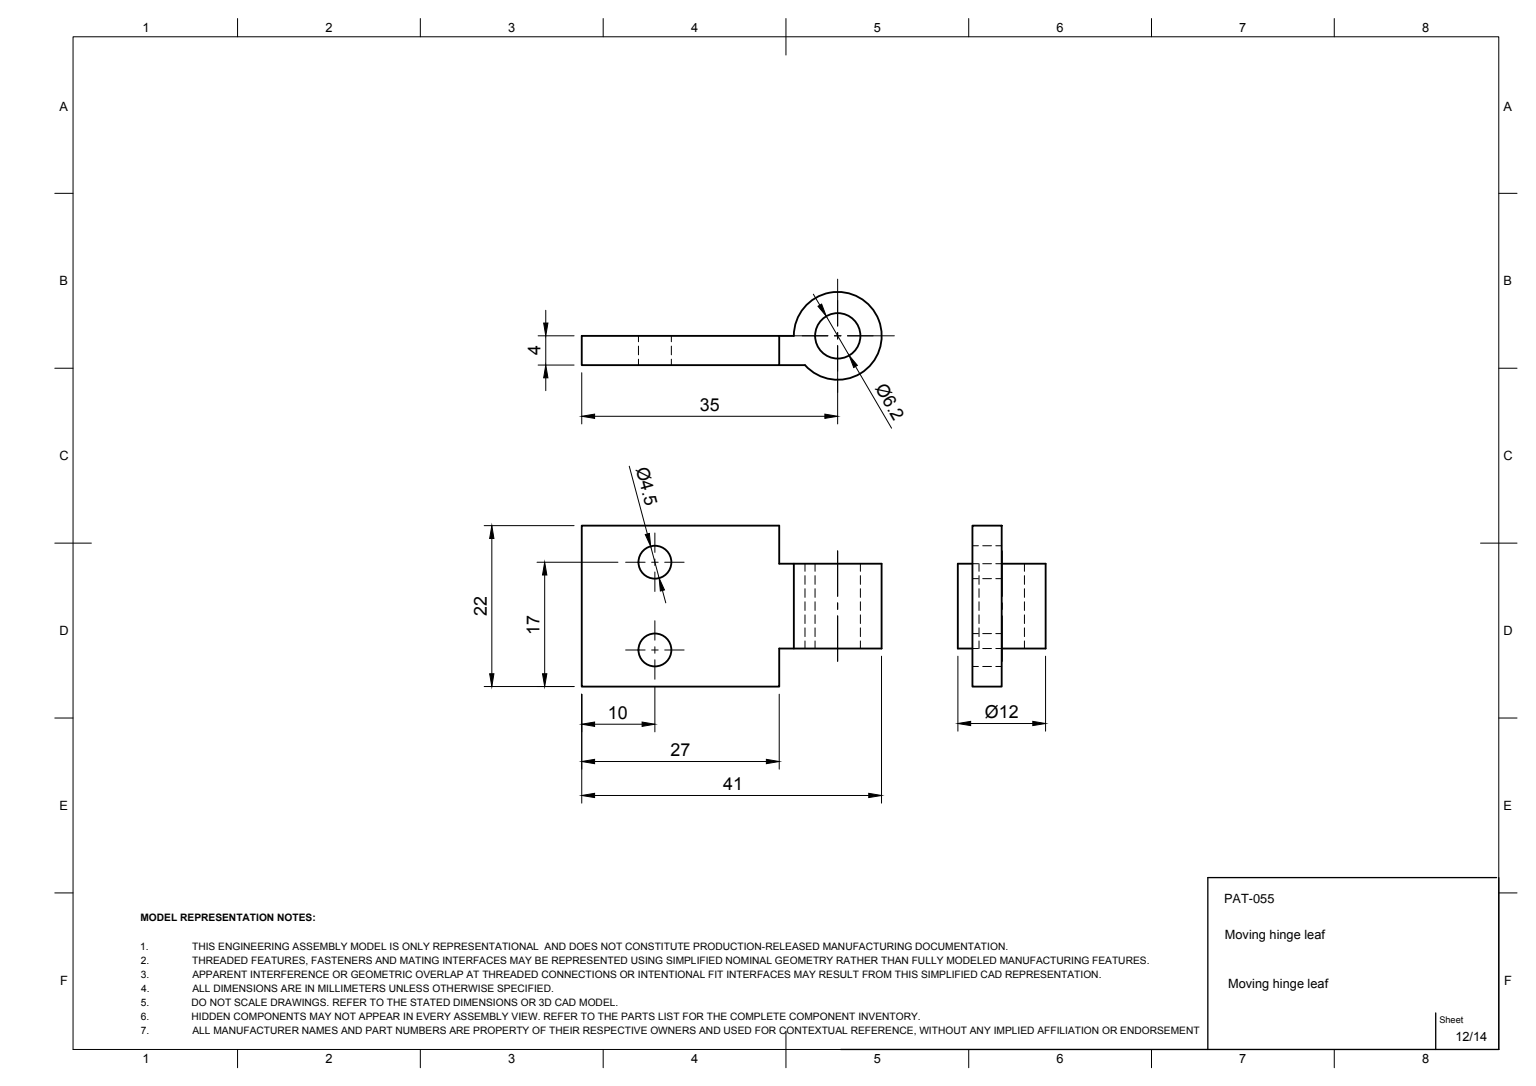
ISO-10303-21;
HEADER;
/* Generated by software containing ST-Developer
 * from STEP Tools, Inc. (www.steptools.com) 
 */

FILE_DESCRIPTION(
/* description */ ('Hinged panel with latch'),
/* implementation_level */ '2;1');

FILE_NAME(
/* name */ 'Moving hinge leaf.step',
/* time_stamp */ '2026-10-27T20:36:01-07:00',
/* author */ (''),
/* organization */ (''),
/* preprocessor_version */ 'ST-DEVELOPER v20.2',
/* originating_system */ 'Autodesk Translation Framework v15.17.0.0',
/* authorisation */ '');

FILE_SCHEMA (('AUTOMOTIVE_DESIGN { 1 0 10303 214 3 1 1 }'));
ENDSEC;

DATA;
#10=MECHANICAL_DESIGN_GEOMETRIC_PRESENTATION_REPRESENTATION('',(#305),#6743);
#273=SHAPE_REPRESENTATION_RELATIONSHIP('SRR','None',#6849,#289);
#289=ADVANCED_BREP_SHAPE_REPRESENTATION('',(#320),#6735);
#305=STYLED_ITEM('',(#6989),#320);
#320=MANIFOLD_SOLID_BREP('Body1',#3808);
#356=FACE_BOUND('',#894,.T.);
#357=FACE_BOUND('',#896,.T.);
#358=FACE_BOUND('',#897,.T.);
#359=FACE_BOUND('',#899,.T.);
#360=FACE_BOUND('',#900,.T.);
#361=FACE_BOUND('',#903,.T.);
#468=PLANE('',#4197);
#469=PLANE('',#4198);
#470=PLANE('',#4199);
#471=PLANE('',#4200);
#472=PLANE('',#4201);
#473=PLANE('',#4202);
#474=PLANE('',#4204);
#475=PLANE('',#4205);
#476=PLANE('',#4208);
#648=FACE_OUTER_BOUND('',#885,.T.);
#649=FACE_OUTER_BOUND('',#886,.T.);
#650=FACE_OUTER_BOUND('',#887,.T.);
#651=FACE_OUTER_BOUND('',#888,.T.);
#652=FACE_OUTER_BOUND('',#889,.T.);
#653=FACE_OUTER_BOUND('',#890,.T.);
#654=FACE_OUTER_BOUND('',#891,.T.);
#655=FACE_OUTER_BOUND('',#892,.T.);
#656=FACE_OUTER_BOUND('',#893,.T.);
#657=FACE_OUTER_BOUND('',#895,.T.);
#658=FACE_OUTER_BOUND('',#898,.T.);
#659=FACE_OUTER_BOUND('',#901,.T.);
#660=FACE_OUTER_BOUND('',#902,.T.);
#885=EDGE_LOOP('',(#3216,#3217,#3218,#3219));
#886=EDGE_LOOP('',(#3220,#3221,#3222,#3223));
#887=EDGE_LOOP('',(#3224,#3225,#3226,#3227));
#888=EDGE_LOOP('',(#3228,#3229,#3230,#3231));
#889=EDGE_LOOP('',(#3232,#3233,#3234,#3235));
#890=EDGE_LOOP('',(#3236,#3237,#3238,#3239));
#891=EDGE_LOOP('',(#3240,#3241,#3242,#3243));
#892=EDGE_LOOP('',(#3244,#3245,#3246,#3247));
#893=EDGE_LOOP('',(#3248,#3249,#3250,#3251));
#894=EDGE_LOOP('',(#3252));
#895=EDGE_LOOP('',(#3253,#3254,#3255,#3256,#3257,#3258,#3259,#3260));
#896=EDGE_LOOP('',(#3261));
#897=EDGE_LOOP('',(#3262));
#898=EDGE_LOOP('',(#3263,#3264,#3265,#3266,#3267,#3268,#3269,#3270));
#899=EDGE_LOOP('',(#3271));
#900=EDGE_LOOP('',(#3272));
#901=EDGE_LOOP('',(#3273,#3274,#3275,#3276));
#902=EDGE_LOOP('',(#3277,#3278,#3279,#3280));
#903=EDGE_LOOP('',(#3281));
#1233=LINE('',#6242,#1591);
#1234=LINE('',#6248,#1592);
#1235=LINE('',#6254,#1593);
#1236=LINE('',#6259,#1594);
#1237=LINE('',#6261,#1595);
#1238=LINE('',#6263,#1596);
#1239=LINE('',#6264,#1597);
#1240=LINE('',#6268,#1598);
#1241=LINE('',#6270,#1599);
#1242=LINE('',#6272,#1600);
#1243=LINE('',#6273,#1601);
#1244=LINE('',#6276,#1602);
#1245=LINE('',#6278,#1603);
#1246=LINE('',#6279,#1604);
#1247=LINE('',#6282,#1605);
#1248=LINE('',#6284,#1606);
#1249=LINE('',#6285,#1607);
#1250=LINE('',#6287,#1608);
#1251=LINE('',#6288,#1609);
#1252=LINE('',#6291,#1610);
#1253=LINE('',#6294,#1611);
#1254=LINE('',#6297,#1612);
#1255=LINE('',#6298,#1613);
#1256=LINE('',#6301,#1614);
#1257=LINE('',#6302,#1615);
#1591=VECTOR('',#5007,0.225);
#1592=VECTOR('',#5014,0.225);
#1593=VECTOR('',#5021,0.31);
#1594=VECTOR('',#5026,1.);
#1595=VECTOR('',#5027,1.);
#1596=VECTOR('',#5028,1.);
#1597=VECTOR('',#5029,1.);
#1598=VECTOR('',#5032,1.);
#1599=VECTOR('',#5033,1.);
#1600=VECTOR('',#5034,1.);
#1601=VECTOR('',#5035,1.);
#1602=VECTOR('',#5038,1.);
#1603=VECTOR('',#5039,1.);
#1604=VECTOR('',#5040,1.);
#1605=VECTOR('',#5043,1.);
#1606=VECTOR('',#5044,1.);
#1607=VECTOR('',#5045,1.);
#1608=VECTOR('',#5048,1.);
#1609=VECTOR('',#5049,1.);
#1610=VECTOR('',#5052,1.);
#1611=VECTOR('',#5055,1.);
#1612=VECTOR('',#5058,1.);
#1613=VECTOR('',#5059,1.);
#1614=VECTOR('',#5062,1.);
#1615=VECTOR('',#5063,1.);
#1752=CIRCLE('',#4189,0.225);
#1753=CIRCLE('',#4190,0.225);
#1754=CIRCLE('',#4192,0.225);
#1755=CIRCLE('',#4193,0.225);
#1756=CIRCLE('',#4195,0.31);
#1757=CIRCLE('',#4196,0.31);
#1758=CIRCLE('',#4203,0.6);
#1759=CIRCLE('',#4207,0.6);
#1998=VERTEX_POINT('',#6239);
#1999=VERTEX_POINT('',#6241);
#2000=VERTEX_POINT('',#6245);
#2001=VERTEX_POINT('',#6247);
#2002=VERTEX_POINT('',#6251);
#2003=VERTEX_POINT('',#6253);
#2004=VERTEX_POINT('',#6257);
#2005=VERTEX_POINT('',#6258);
#2006=VERTEX_POINT('',#6260);
#2007=VERTEX_POINT('',#6262);
#2008=VERTEX_POINT('',#6266);
#2009=VERTEX_POINT('',#6267);
#2010=VERTEX_POINT('',#6269);
#2011=VERTEX_POINT('',#6271);
#2012=VERTEX_POINT('',#6275);
#2013=VERTEX_POINT('',#6277);
#2014=VERTEX_POINT('',#6281);
#2015=VERTEX_POINT('',#6283);
#2016=VERTEX_POINT('',#6290);
#2017=VERTEX_POINT('',#6292);
#2018=VERTEX_POINT('',#6296);
#2019=VERTEX_POINT('',#6300);
#2420=EDGE_CURVE('',#1998,#1998,#1752,.T.);
#2421=EDGE_CURVE('',#1998,#1999,#1233,.T.);
#2422=EDGE_CURVE('',#1999,#1999,#1753,.T.);
#2423=EDGE_CURVE('',#2000,#2000,#1754,.T.);
#2424=EDGE_CURVE('',#2000,#2001,#1234,.T.);
#2425=EDGE_CURVE('',#2001,#2001,#1755,.T.);
#2426=EDGE_CURVE('',#2002,#2002,#1756,.T.);
#2427=EDGE_CURVE('',#2002,#2003,#1235,.T.);
#2428=EDGE_CURVE('',#2003,#2003,#1757,.T.);
#2429=EDGE_CURVE('',#2004,#2005,#1236,.T.);
#2430=EDGE_CURVE('',#2006,#2004,#1237,.T.);
#2431=EDGE_CURVE('',#2006,#2007,#1238,.T.);
#2432=EDGE_CURVE('',#2005,#2007,#1239,.T.);
#2433=EDGE_CURVE('',#2008,#2009,#1240,.T.);
#2434=EDGE_CURVE('',#2010,#2008,#1241,.T.);
#2435=EDGE_CURVE('',#2011,#2010,#1242,.T.);
#2436=EDGE_CURVE('',#2009,#2011,#1243,.T.);
#2437=EDGE_CURVE('',#2011,#2012,#1244,.T.);
#2438=EDGE_CURVE('',#2013,#2010,#1245,.T.);
#2439=EDGE_CURVE('',#2012,#2013,#1246,.T.);
#2440=EDGE_CURVE('',#2012,#2014,#1247,.T.);
#2441=EDGE_CURVE('',#2015,#2013,#1248,.T.);
#2442=EDGE_CURVE('',#2014,#2015,#1249,.T.);
#2443=EDGE_CURVE('',#2014,#2006,#1250,.T.);
#2444=EDGE_CURVE('',#2007,#2015,#1251,.T.);
#2445=EDGE_CURVE('',#2016,#2009,#1252,.T.);
#2446=EDGE_CURVE('',#2017,#2016,#1758,.T.);
#2447=EDGE_CURVE('',#2008,#2017,#1253,.T.);
#2448=EDGE_CURVE('',#2004,#2018,#1254,.T.);
#2449=EDGE_CURVE('',#2016,#2018,#1255,.T.);
#2450=EDGE_CURVE('',#2019,#2017,#1256,.T.);
#2451=EDGE_CURVE('',#2019,#2005,#1257,.T.);
#2452=EDGE_CURVE('',#2019,#2018,#1759,.T.);
#3216=ORIENTED_EDGE('',*,*,#2420,.F.);
#3217=ORIENTED_EDGE('',*,*,#2421,.T.);
#3218=ORIENTED_EDGE('',*,*,#2422,.F.);
#3219=ORIENTED_EDGE('',*,*,#2421,.F.);
#3220=ORIENTED_EDGE('',*,*,#2423,.F.);
#3221=ORIENTED_EDGE('',*,*,#2424,.T.);
#3222=ORIENTED_EDGE('',*,*,#2425,.F.);
#3223=ORIENTED_EDGE('',*,*,#2424,.F.);
#3224=ORIENTED_EDGE('',*,*,#2426,.F.);
#3225=ORIENTED_EDGE('',*,*,#2427,.T.);
#3226=ORIENTED_EDGE('',*,*,#2428,.F.);
#3227=ORIENTED_EDGE('',*,*,#2427,.F.);
#3228=ORIENTED_EDGE('',*,*,#2429,.F.);
#3229=ORIENTED_EDGE('',*,*,#2430,.F.);
#3230=ORIENTED_EDGE('',*,*,#2431,.T.);
#3231=ORIENTED_EDGE('',*,*,#2432,.F.);
#3232=ORIENTED_EDGE('',*,*,#2433,.F.);
#3233=ORIENTED_EDGE('',*,*,#2434,.F.);
#3234=ORIENTED_EDGE('',*,*,#2435,.F.);
#3235=ORIENTED_EDGE('',*,*,#2436,.F.);
#3236=ORIENTED_EDGE('',*,*,#2437,.F.);
#3237=ORIENTED_EDGE('',*,*,#2435,.T.);
#3238=ORIENTED_EDGE('',*,*,#2438,.F.);
#3239=ORIENTED_EDGE('',*,*,#2439,.F.);
#3240=ORIENTED_EDGE('',*,*,#2440,.F.);
#3241=ORIENTED_EDGE('',*,*,#2439,.T.);
#3242=ORIENTED_EDGE('',*,*,#2441,.F.);
#3243=ORIENTED_EDGE('',*,*,#2442,.F.);
#3244=ORIENTED_EDGE('',*,*,#2443,.F.);
#3245=ORIENTED_EDGE('',*,*,#2442,.T.);
#3246=ORIENTED_EDGE('',*,*,#2444,.F.);
#3247=ORIENTED_EDGE('',*,*,#2431,.F.);
#3248=ORIENTED_EDGE('',*,*,#2433,.T.);
#3249=ORIENTED_EDGE('',*,*,#2445,.F.);
#3250=ORIENTED_EDGE('',*,*,#2446,.F.);
#3251=ORIENTED_EDGE('',*,*,#2447,.F.);
#3252=ORIENTED_EDGE('',*,*,#2426,.T.);
#3253=ORIENTED_EDGE('',*,*,#2448,.T.);
#3254=ORIENTED_EDGE('',*,*,#2449,.F.);
#3255=ORIENTED_EDGE('',*,*,#2445,.T.);
#3256=ORIENTED_EDGE('',*,*,#2436,.T.);
#3257=ORIENTED_EDGE('',*,*,#2437,.T.);
#3258=ORIENTED_EDGE('',*,*,#2440,.T.);
#3259=ORIENTED_EDGE('',*,*,#2443,.T.);
#3260=ORIENTED_EDGE('',*,*,#2430,.T.);
#3261=ORIENTED_EDGE('',*,*,#2420,.T.);
#3262=ORIENTED_EDGE('',*,*,#2423,.T.);
#3263=ORIENTED_EDGE('',*,*,#2447,.T.);
#3264=ORIENTED_EDGE('',*,*,#2450,.F.);
#3265=ORIENTED_EDGE('',*,*,#2451,.T.);
#3266=ORIENTED_EDGE('',*,*,#2432,.T.);
#3267=ORIENTED_EDGE('',*,*,#2444,.T.);
#3268=ORIENTED_EDGE('',*,*,#2441,.T.);
#3269=ORIENTED_EDGE('',*,*,#2438,.T.);
#3270=ORIENTED_EDGE('',*,*,#2434,.T.);
#3271=ORIENTED_EDGE('',*,*,#2422,.T.);
#3272=ORIENTED_EDGE('',*,*,#2425,.T.);
#3273=ORIENTED_EDGE('',*,*,#2449,.T.);
#3274=ORIENTED_EDGE('',*,*,#2452,.F.);
#3275=ORIENTED_EDGE('',*,*,#2450,.T.);
#3276=ORIENTED_EDGE('',*,*,#2446,.T.);
#3277=ORIENTED_EDGE('',*,*,#2429,.T.);
#3278=ORIENTED_EDGE('',*,*,#2451,.F.);
#3279=ORIENTED_EDGE('',*,*,#2452,.T.);
#3280=ORIENTED_EDGE('',*,*,#2448,.F.);
#3281=ORIENTED_EDGE('',*,*,#2428,.T.);
#3579=CYLINDRICAL_SURFACE('',#4188,0.225);
#3580=CYLINDRICAL_SURFACE('',#4191,0.225);
#3581=CYLINDRICAL_SURFACE('',#4194,0.31);
#3582=CYLINDRICAL_SURFACE('',#4206,0.6);
#3717=ADVANCED_FACE('',(#648),#3579,.F.);
#3718=ADVANCED_FACE('',(#649),#3580,.F.);
#3719=ADVANCED_FACE('',(#650),#3581,.F.);
#3720=ADVANCED_FACE('',(#651),#468,.T.);
#3721=ADVANCED_FACE('',(#652),#469,.T.);
#3722=ADVANCED_FACE('',(#653),#470,.T.);
#3723=ADVANCED_FACE('',(#654),#471,.T.);
#3724=ADVANCED_FACE('',(#655),#472,.T.);
#3725=ADVANCED_FACE('',(#656,#356),#473,.F.);
#3726=ADVANCED_FACE('',(#657,#357,#358),#474,.F.);
#3727=ADVANCED_FACE('',(#658,#359,#360),#475,.T.);
#3728=ADVANCED_FACE('',(#659),#3582,.T.);
#3729=ADVANCED_FACE('',(#660,#361),#476,.T.);
#3808=CLOSED_SHELL('',(#3717,#3718,#3719,#3720,#3721,#3722,#3723,#3724,
#3725,#3726,#3727,#3728,#3729));
#4187=AXIS2_PLACEMENT_3D('',#6237,#5001,#5002);
#4188=AXIS2_PLACEMENT_3D('',#6238,#5003,#5004);
#4189=AXIS2_PLACEMENT_3D('',#6240,#5005,#5006);
#4190=AXIS2_PLACEMENT_3D('',#6243,#5008,#5009);
#4191=AXIS2_PLACEMENT_3D('',#6244,#5010,#5011);
#4192=AXIS2_PLACEMENT_3D('',#6246,#5012,#5013);
#4193=AXIS2_PLACEMENT_3D('',#6249,#5015,#5016);
#4194=AXIS2_PLACEMENT_3D('',#6250,#5017,#5018);
#4195=AXIS2_PLACEMENT_3D('',#6252,#5019,#5020);
#4196=AXIS2_PLACEMENT_3D('',#6255,#5022,#5023);
#4197=AXIS2_PLACEMENT_3D('',#6256,#5024,#5025);
#4198=AXIS2_PLACEMENT_3D('',#6265,#5030,#5031);
#4199=AXIS2_PLACEMENT_3D('',#6274,#5036,#5037);
#4200=AXIS2_PLACEMENT_3D('',#6280,#5041,#5042);
#4201=AXIS2_PLACEMENT_3D('',#6286,#5046,#5047);
#4202=AXIS2_PLACEMENT_3D('',#6289,#5050,#5051);
#4203=AXIS2_PLACEMENT_3D('',#6293,#5053,#5054);
#4204=AXIS2_PLACEMENT_3D('',#6295,#5056,#5057);
#4205=AXIS2_PLACEMENT_3D('',#6299,#5060,#5061);
#4206=AXIS2_PLACEMENT_3D('',#6303,#5064,#5065);
#4207=AXIS2_PLACEMENT_3D('',#6304,#5066,#5067);
#4208=AXIS2_PLACEMENT_3D('',#6305,#5068,#5069);
#5001=DIRECTION('axis',(0.,0.,1.));
#5002=DIRECTION('refdir',(1.,0.,0.));
#5003=DIRECTION('center_axis',(0.,1.,0.));
#5004=DIRECTION('ref_axis',(1.,0.,0.));
#5005=DIRECTION('center_axis',(0.,1.,0.));
#5006=DIRECTION('ref_axis',(1.,0.,0.));
#5007=DIRECTION('',(0.,1.,0.));
#5008=DIRECTION('center_axis',(0.,-1.,0.));
#5009=DIRECTION('ref_axis',(1.,0.,0.));
#5010=DIRECTION('center_axis',(0.,1.,0.));
#5011=DIRECTION('ref_axis',(1.,0.,0.));
#5012=DIRECTION('center_axis',(0.,1.,0.));
#5013=DIRECTION('ref_axis',(1.,0.,0.));
#5014=DIRECTION('',(0.,1.,0.));
#5015=DIRECTION('center_axis',(0.,-1.,0.));
#5016=DIRECTION('ref_axis',(1.,0.,0.));
#5017=DIRECTION('center_axis',(0.,0.,1.));
#5018=DIRECTION('ref_axis',(1.,0.,0.));
#5019=DIRECTION('center_axis',(0.,0.,1.));
#5020=DIRECTION('ref_axis',(1.,0.,0.));
#5021=DIRECTION('',(0.,0.,1.));
#5022=DIRECTION('center_axis',(0.,0.,-1.));
#5023=DIRECTION('ref_axis',(1.,0.,0.));
#5024=DIRECTION('center_axis',(-1.,0.,0.));
#5025=DIRECTION('ref_axis',(0.,0.,1.));
#5026=DIRECTION('',(0.,1.,0.));
#5027=DIRECTION('',(0.,0.,-1.));
#5028=DIRECTION('',(0.,1.,0.));
#5029=DIRECTION('',(0.,0.,1.));
#5030=DIRECTION('center_axis',(-1.,0.,0.));
#5031=DIRECTION('ref_axis',(0.,0.,1.));
#5032=DIRECTION('',(0.,-1.,0.));
#5033=DIRECTION('',(0.,0.,1.));
#5034=DIRECTION('',(0.,1.,0.));
#5035=DIRECTION('',(0.,0.,-1.));
#5036=DIRECTION('center_axis',(0.,0.,-1.));
#5037=DIRECTION('ref_axis',(-1.,0.,0.));
#5038=DIRECTION('',(1.,0.,0.));
#5039=DIRECTION('',(-1.,0.,0.));
#5040=DIRECTION('',(0.,1.,0.));
#5041=DIRECTION('center_axis',(1.,0.,0.));
#5042=DIRECTION('ref_axis',(0.,0.,-1.));
#5043=DIRECTION('',(0.,0.,1.));
#5044=DIRECTION('',(0.,0.,-1.));
#5045=DIRECTION('',(0.,1.,0.));
#5046=DIRECTION('center_axis',(0.,0.,1.));
#5047=DIRECTION('ref_axis',(1.,0.,0.));
#5048=DIRECTION('',(-1.,0.,0.));
#5049=DIRECTION('',(1.,0.,0.));
#5050=DIRECTION('center_axis',(0.,0.,1.));
#5051=DIRECTION('ref_axis',(1.,0.,0.));
#5052=DIRECTION('',(1.,0.,0.));
#5053=DIRECTION('center_axis',(0.,0.,1.));
#5054=DIRECTION('ref_axis',(1.,0.,0.));
#5055=DIRECTION('',(-1.,0.,0.));
#5056=DIRECTION('center_axis',(0.,1.,0.));
#5057=DIRECTION('ref_axis',(1.,0.,0.));
#5058=DIRECTION('',(-1.,0.,0.));
#5059=DIRECTION('',(0.,0.,1.));
#5060=DIRECTION('center_axis',(0.,1.,0.));
#5061=DIRECTION('ref_axis',(0.,0.,1.));
#5062=DIRECTION('',(0.,0.,-1.));
#5063=DIRECTION('',(1.,0.,0.));
#5064=DIRECTION('center_axis',(0.,0.,1.));
#5065=DIRECTION('ref_axis',(-0.934172358962716,0.35682208977309,0.));
#5066=DIRECTION('center_axis',(0.,0.,1.));
#5067=DIRECTION('ref_axis',(1.,0.,0.));
#5068=DIRECTION('center_axis',(0.,0.,1.));
#5069=DIRECTION('ref_axis',(1.,0.,0.));
#6237=CARTESIAN_POINT('',(0.,0.,0.));
#6238=CARTESIAN_POINT('Origin',(4.5,-2.3,6.));
#6239=CARTESIAN_POINT('',(4.275,-2.2,6.));
#6240=CARTESIAN_POINT('Origin',(4.5,-2.2,6.));
#6241=CARTESIAN_POINT('',(4.275,-1.8,6.));
#6242=CARTESIAN_POINT('',(4.275,-2.3,6.));
#6243=CARTESIAN_POINT('Origin',(4.5,-1.8,6.));
#6244=CARTESIAN_POINT('Origin',(4.5,-2.3,7.2));
#6245=CARTESIAN_POINT('',(4.275,-2.2,7.2));
#6246=CARTESIAN_POINT('Origin',(4.5,-2.2,7.2));
#6247=CARTESIAN_POINT('',(4.275,-1.8,7.2));
#6248=CARTESIAN_POINT('',(4.275,-2.3,7.2));
#6249=CARTESIAN_POINT('Origin',(4.5,-1.8,7.2));
#6250=CARTESIAN_POINT('Origin',(2.,-1.8,6.));
#6251=CARTESIAN_POINT('',(1.69,-1.8,6.02));
#6252=CARTESIAN_POINT('Origin',(2.,-1.8,6.02));
#6253=CARTESIAN_POINT('',(1.69,-1.8,7.18));
#6254=CARTESIAN_POINT('',(1.69,-1.8,6.));
#6255=CARTESIAN_POINT('Origin',(2.,-1.8,7.18));
#6256=CARTESIAN_POINT('Origin',(2.8,-2.2,5.5));
#6257=CARTESIAN_POINT('',(2.8,-2.2,7.18));
#6258=CARTESIAN_POINT('',(2.8,-1.8,7.18));
#6259=CARTESIAN_POINT('',(2.8,-2.,7.18));
#6260=CARTESIAN_POINT('',(2.8,-2.2,7.7));
#6261=CARTESIAN_POINT('',(2.8,-2.2,7.7));
#6262=CARTESIAN_POINT('',(2.8,-1.8,7.7));
#6263=CARTESIAN_POINT('',(2.8,-2.2,7.7));
#6264=CARTESIAN_POINT('',(2.8,-1.8,7.7));
#6265=CARTESIAN_POINT('Origin',(2.8,-2.2,5.5));
#6266=CARTESIAN_POINT('',(2.8,-1.8,6.02));
#6267=CARTESIAN_POINT('',(2.8,-2.2,6.02));
#6268=CARTESIAN_POINT('',(2.8,-2.,6.02));
#6269=CARTESIAN_POINT('',(2.8,-1.8,5.5));
#6270=CARTESIAN_POINT('',(2.8,-1.8,7.7));
#6271=CARTESIAN_POINT('',(2.8,-2.2,5.5));
#6272=CARTESIAN_POINT('',(2.8,-2.2,5.5));
#6273=CARTESIAN_POINT('',(2.8,-2.2,7.7));
#6274=CARTESIAN_POINT('Origin',(5.5,-2.2,5.5));
#6275=CARTESIAN_POINT('',(5.5,-2.2,5.5));
#6276=CARTESIAN_POINT('',(2.8,-2.2,5.5));
#6277=CARTESIAN_POINT('',(5.5,-1.8,5.5));
#6278=CARTESIAN_POINT('',(2.8,-1.8,5.5));
#6279=CARTESIAN_POINT('',(5.5,-2.2,5.5));
#6280=CARTESIAN_POINT('Origin',(5.5,-2.2,7.7));
#6281=CARTESIAN_POINT('',(5.5,-2.2,7.7));
#6282=CARTESIAN_POINT('',(5.5,-2.2,5.5));
#6283=CARTESIAN_POINT('',(5.5,-1.8,7.7));
#6284=CARTESIAN_POINT('',(5.5,-1.8,5.5));
#6285=CARTESIAN_POINT('',(5.5,-2.2,7.7));
#6286=CARTESIAN_POINT('Origin',(2.8,-2.2,7.7));
#6287=CARTESIAN_POINT('',(5.5,-2.2,7.7));
#6288=CARTESIAN_POINT('',(5.5,-1.8,7.7));
#6289=CARTESIAN_POINT('Origin',(2.,-1.8,6.02));
#6290=CARTESIAN_POINT('',(2.44721359549996,-2.2,6.02));
#6291=CARTESIAN_POINT('',(2.,-2.2,6.02));
#6292=CARTESIAN_POINT('',(2.6,-1.8,6.02));
#6293=CARTESIAN_POINT('Origin',(2.,-1.8,6.02));
#6294=CARTESIAN_POINT('',(2.,-1.8,6.02));
#6295=CARTESIAN_POINT('Origin',(2.5,-2.2,6.6));
#6296=CARTESIAN_POINT('',(2.44721359549996,-2.2,7.18));
#6297=CARTESIAN_POINT('',(3.,-2.2,7.18));
#6298=CARTESIAN_POINT('',(2.44721359549996,-2.2,6.02));
#6299=CARTESIAN_POINT('Origin',(2.5,-1.8,6.6));
#6300=CARTESIAN_POINT('',(2.6,-1.8,7.18));
#6301=CARTESIAN_POINT('',(2.6,-1.8,6.02));
#6302=CARTESIAN_POINT('',(3.,-1.8,7.18));
#6303=CARTESIAN_POINT('Origin',(2.,-1.8,6.02));
#6304=CARTESIAN_POINT('Origin',(2.,-1.8,7.18));
#6305=CARTESIAN_POINT('Origin',(2.,-1.8,7.18));
#6714=UNCERTAINTY_MEASURE_WITH_UNIT(LENGTH_MEASURE(0.001),#6744,
'DISTANCE_ACCURACY_VALUE',
'Maximum model space distance between geometric entities at asserted c
onnectivities');
#6722=UNCERTAINTY_MEASURE_WITH_UNIT(LENGTH_MEASURE(0.001),#6744,
'DISTANCE_ACCURACY_VALUE',
'Maximum model space distance between geometric entities at asserted c
onnectivities');
#6735=(
GEOMETRIC_REPRESENTATION_CONTEXT(3)
GLOBAL_UNCERTAINTY_ASSIGNED_CONTEXT((#6714))
GLOBAL_UNIT_ASSIGNED_CONTEXT((#6744,#6746,#6747))
REPRESENTATION_CONTEXT('','3D')
);
#6743=(
GEOMETRIC_REPRESENTATION_CONTEXT(3)
GLOBAL_UNCERTAINTY_ASSIGNED_CONTEXT((#6722))
GLOBAL_UNIT_ASSIGNED_CONTEXT((#6744,#6746,#6747))
REPRESENTATION_CONTEXT('','3D')
);
#6744=(
LENGTH_UNIT()
NAMED_UNIT(*)
SI_UNIT(.CENTI.,.METRE.)
);
#6746=(
NAMED_UNIT(*)
PLANE_ANGLE_UNIT()
SI_UNIT($,.RADIAN.)
);
#6747=(
NAMED_UNIT(*)
SI_UNIT($,.STERADIAN.)
SOLID_ANGLE_UNIT()
);
#6760=SHAPE_DEFINITION_REPRESENTATION(#6780,#6849);
#6780=PRODUCT_DEFINITION_SHAPE('',$,#6870);
#6849=SHAPE_REPRESENTATION('',(#4187),#6735);
#6857=PRODUCT_DEFINITION_CONTEXT('part definition',#6919,'design');
#6870=PRODUCT_DEFINITION('Moving hinge leaf','Moving hinge leaf',#6890,
#6857);
#6890=PRODUCT_DEFINITION_FORMATION('',$,#6933);
#6919=APPLICATION_CONTEXT(
'Core Data for Automotive Mechanical Design Process');
#6920=PRODUCT_CONTEXT('part definition',#6919,'mechanical');
#6933=PRODUCT('Moving hinge leaf','Moving hinge leaf',
'Moving hinge leaf',(#6920));
#6983=COLOUR_RGB('Light Blue',0.38,0.62,0.78);
#6984=FILL_AREA_STYLE_COLOUR('',#6983);
#6985=FILL_AREA_STYLE('',(#6984));
#6986=SURFACE_STYLE_FILL_AREA(#6985);
#6987=SURFACE_SIDE_STYLE('',(#6986));
#6988=SURFACE_STYLE_USAGE(.BOTH.,#6987);
#6989=PRESENTATION_STYLE_ASSIGNMENT((#6988));
ENDSEC;
END-ISO-10303-21;
